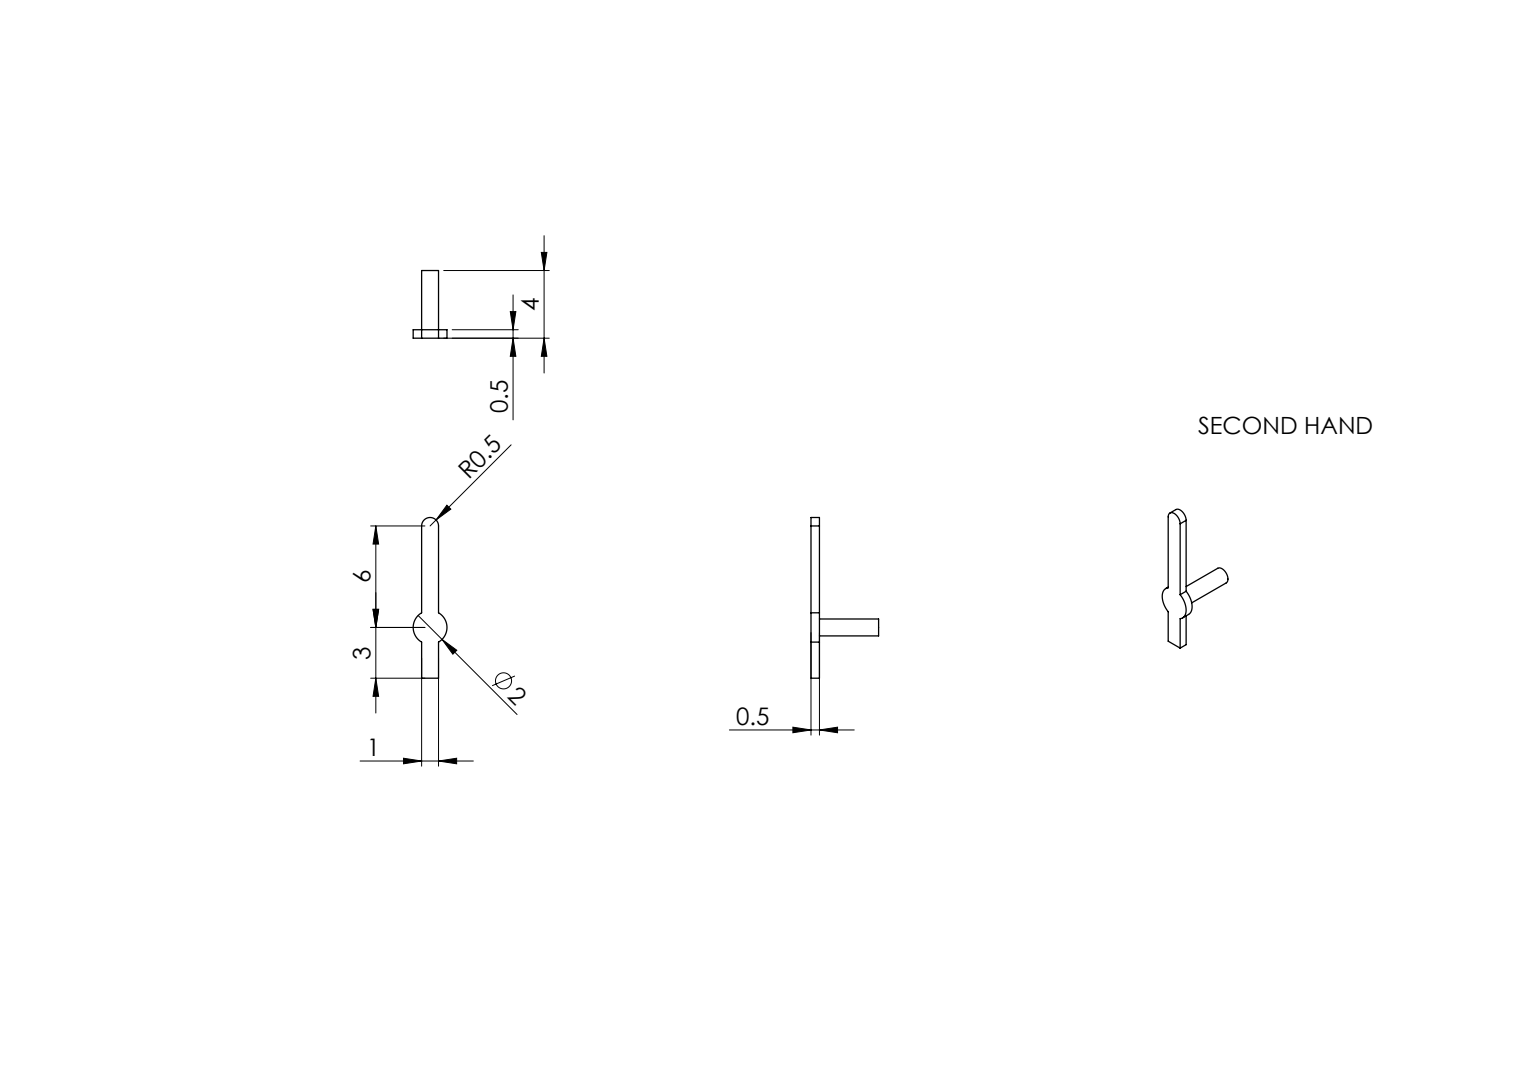
ISO-10303-21;
HEADER;
FILE_DESCRIPTION (('STEP AP214'),
    '1' );
FILE_NAME ('second hand.step',
    '2026-10-26T11:20:31',
    ( '' ),
    ( '' ),
    'SwSTEP 2.0',
    'SolidWorks 2026',
    '' );
FILE_SCHEMA (( 'AUTOMOTIVE_DESIGN' ));
ENDSEC;

DATA;
#9=FACE_OUTER_BOUND ( 'NONE', #3478, .T. ) ;
#19=CARTESIAN_POINT ( 'NONE',  ( -0.5000000000000000000, -2.999999999999999556, 19.50000000000000000 ) ) ;
#36=AXIS2_PLACEMENT_3D ( 'NONE', #4466, #800, #1180 ) ;
#37=CARTESIAN_POINT ( 'NONE',  ( 0.5000000000000001110, 6.123233995736767268E-17, 20.00000000000000000 ) ) ;
#46=ORIENTED_EDGE ( 'NONE', *, *, #3772, .T. ) ;
#54=EDGE_CURVE ( 'NONE', #3353, #742, #2591, .T. ) ;
#56=DIRECTION ( 'NONE',  ( 1.000000000000000000, 0.000000000000000000, -0.000000000000000000 ) ) ;
#58=CARTESIAN_POINT ( 'NONE',  ( -0.5000000000000000000, 0.000000000000000000, 20.00000000000000000 ) ) ;
#60=ORIENTED_EDGE ( 'NONE', *, *, #514, .T. ) ;
#93=PLANE ( 'NONE',  #36 ) ;
#95=ORIENTED_EDGE ( 'NONE', *, *, #3675, .F. ) ;
#128=CARTESIAN_POINT ( 'NONE',  ( -0.5000000000000000000, -2.999999999999999556, 20.00000000000000000 ) ) ;
#137=DIRECTION ( 'NONE',  ( 0.000000000000000000, 0.000000000000000000, 1.000000000000000000 ) ) ;
#163=DIRECTION ( 'NONE',  ( -0.000000000000000000, -1.000000000000000000, 0.000000000000000000 ) ) ;
#177=VERTEX_POINT ( 'NONE', #3882 ) ;
#192=ORIENTED_EDGE ( 'NONE', *, *, #766, .F. ) ;
#197=VECTOR ( 'NONE', #3332, 1000.000000000000000 ) ;
#198=EDGE_CURVE ( 'NONE', #954, #442, #3903, .T. ) ;
#199=EDGE_CURVE ( 'NONE', #177, #2707, #3976, .T. ) ;
#209=CARTESIAN_POINT ( 'NONE',  ( 1.000000000000000000, 0.000000000000000000, 20.00000000000000000 ) ) ;
#216=ORIENTED_EDGE ( 'NONE', *, *, #4488, .T. ) ;
#225=AXIS2_PLACEMENT_3D ( 'NONE', #2885, #1132, #2148 ) ;
#232=CARTESIAN_POINT ( 'NONE',  ( -0.5000000000000000000, 0.000000000000000000, 19.50000000000000000 ) ) ;
#249=ORIENTED_EDGE ( 'NONE', *, *, #4128, .F. ) ;
#252=PLANE ( 'NONE',  #505 ) ;
#279=LINE ( 'NONE', #643, #686 ) ;
#281=EDGE_CURVE ( 'NONE', #1290, #3612, #2017, .T. ) ;
#296=AXIS2_PLACEMENT_3D ( 'NONE', #2408, #3159, #4617 ) ;
#302=CARTESIAN_POINT ( 'NONE',  ( 0.000000000000000000, 0.000000000000000000, 16.00000000000000000 ) ) ;
#312=ADVANCED_FACE ( 'NONE', ( #2776 ), #4236, .F. ) ;
#322=AXIS2_PLACEMENT_3D ( 'NONE', #4183, #3766, #484 ) ;
#326=EDGE_LOOP ( 'NONE', ( #3897, #833, #3483, #60 ) ) ;
#329=SURFACE_SIDE_STYLE ('',( #2159 ) ) ;
#330=DIRECTION ( 'NONE',  ( -1.000000000000000000, 0.000000000000000000, -0.000000000000000000 ) ) ;
#337=AXIS2_PLACEMENT_3D ( 'NONE', #302, #2550, #4345 ) ;
#348=CARTESIAN_POINT ( 'NONE',  ( -0.5000000000000000000, -0.8660254037844387076, 19.50000000000000000 ) ) ;
#355=ORIENTED_EDGE ( 'NONE', *, *, #1156, .F. ) ;
#375=DIRECTION ( 'NONE',  ( 0.000000000000000000, 0.000000000000000000, 1.000000000000000000 ) ) ;
#382=FACE_OUTER_BOUND ( 'NONE', #909, .T. ) ;
#384=CARTESIAN_POINT ( 'NONE',  ( 0.5000000000000000000, 0.000000000000000000, 19.50000000000000000 ) ) ;
#404=SHAPE_REPRESENTATION ( 'second hand', ( #2928 ), #3465 ) ;
#423=CYLINDRICAL_SURFACE ( 'NONE', #4197, 1.000000000000000000 ) ;
#424=EDGE_LOOP ( 'NONE', ( #1754, #498 ) ) ;
#434=ORIENTED_EDGE ( 'NONE', *, *, #4128, .T. ) ;
#442=VERTEX_POINT ( 'NONE', #348 ) ;
#454=CARTESIAN_POINT ( 'NONE',  ( -0.5000000000000001110, 0.000000000000000000, 16.00000000000000000 ) ) ;
#461=CARTESIAN_POINT ( 'NONE',  ( -0.5000000000000000000, 6.000000000000000000, 19.50000000000000000 ) ) ;
#464=CARTESIAN_POINT ( 'NONE',  ( 0.5000000000000000000, -2.999999999999999556, 19.50000000000000000 ) ) ;
#466=DIRECTION ( 'NONE',  ( 1.000000000000000000, 0.000000000000000000, -0.000000000000000000 ) ) ;
#472=VECTOR ( 'NONE', #1598, 1000.000000000000000 ) ;
#474=FACE_OUTER_BOUND ( 'NONE', #326, .T. ) ;
#484=DIRECTION ( 'NONE',  ( 1.000000000000000000, 0.000000000000000000, 0.000000000000000000 ) ) ;
#498=ORIENTED_EDGE ( 'NONE', *, *, #3330, .T. ) ;
#499=VERTEX_POINT ( 'NONE', #19 ) ;
#505=AXIS2_PLACEMENT_3D ( 'NONE', #4213, #3849, #899 ) ;
#514=EDGE_CURVE ( 'NONE', #3612, #442, #4534, .T. ) ;
#527=VECTOR ( 'NONE', #1706, 1000.000000000000000 ) ;
#553=CIRCLE ( 'NONE', #2066, 1.000000000000000000 ) ;
#555=( NAMED_UNIT ( * ) SI_UNIT ( $, .STERADIAN. ) SOLID_ANGLE_UNIT ( ) );
#557=VECTOR ( 'NONE', #4315, 1000.000000000000000 ) ;
#575=LINE ( 'NONE', #4261, #2798 ) ;
#603=ADVANCED_FACE ( 'NONE', ( #1206 ), #2987, .F. ) ;
#643=CARTESIAN_POINT ( 'NONE',  ( 0.5000000000000000000, 0.000000000000000000, 20.00000000000000000 ) ) ;
#654=DIRECTION ( 'NONE',  ( 0.000000000000000000, 0.000000000000000000, 1.000000000000000000 ) ) ;
#673=DIRECTION ( 'NONE',  ( -0.000000000000000000, 0.000000000000000000, 1.000000000000000000 ) ) ;
#686=VECTOR ( 'NONE', #1993, 1000.000000000000000 ) ;
#689=FACE_OUTER_BOUND ( 'NONE', #2400, .T. ) ;
#691=DIRECTION ( 'NONE',  ( 1.000000000000000000, 0.000000000000000000, 0.000000000000000000 ) ) ;
#725=CARTESIAN_POINT ( 'NONE',  ( -0.5000000000000000000, 0.000000000000000000, 19.50000000000000000 ) ) ;
#726=DIRECTION ( 'NONE',  ( 1.000000000000000000, 0.000000000000000000, 0.000000000000000000 ) ) ;
#727=EDGE_CURVE ( 'NONE', #442, #499, #2378, .T. ) ;
#736=ORIENTED_EDGE ( 'NONE', *, *, #2437, .F. ) ;
#737=EDGE_LOOP ( 'NONE', ( #3427, #3754, #3126, #2585 ) ) ;
#742=VERTEX_POINT ( 'NONE', #209 ) ;
#751=EDGE_CURVE ( 'NONE', #954, #2636, #2353, .T. ) ;
#766=EDGE_CURVE ( 'NONE', #1507, #1468, #1480, .T. ) ;
#791=CARTESIAN_POINT ( 'NONE',  ( 0.000000000000000000, 6.000000000000000000, 19.50000000000000000 ) ) ;
#792=CARTESIAN_POINT ( 'NONE',  ( 0.5000000000000001110, 6.123233995736767268E-17, 16.00000000000000000 ) ) ;
#795=PLANE ( 'NONE',  #1205 ) ;
#798=MECHANICAL_DESIGN_GEOMETRIC_PRESENTATION_REPRESENTATION('',(#3759),#4070);
#800=DIRECTION ( 'NONE',  ( 0.000000000000000000, 0.000000000000000000, 1.000000000000000000 ) ) ;
#803=VERTEX_POINT ( 'NONE', #3872 ) ;
#807=ADVANCED_FACE ( 'NONE', ( #2697 ), #252, .T. ) ;
#818=DIRECTION ( 'NONE',  ( -0.000000000000000000, -0.000000000000000000, -1.000000000000000000 ) ) ;
#831=CARTESIAN_POINT ( 'NONE',  ( 0.000000000000000000, 0.000000000000000000, 19.50000000000000000 ) ) ;
#832=CARTESIAN_POINT ( 'NONE',  ( 0.5000000000000000000, 0.000000000000000000, 19.50000000000000000 ) ) ;
#833=ORIENTED_EDGE ( 'NONE', *, *, #2217, .F. ) ;
#841=LINE ( 'NONE', #58, #197 ) ;
#861=AXIS2_PLACEMENT_3D ( 'NONE', #1053, #2489, #4334 ) ;
#862=DIRECTION ( 'NONE',  ( 0.000000000000000000, 0.000000000000000000, 1.000000000000000000 ) ) ;
#892=LINE ( 'NONE', #4485, #4501 ) ;
#895=VERTEX_POINT ( 'NONE', #792 ) ;
#899=DIRECTION ( 'NONE',  ( -0.000000000000000000, 0.000000000000000000, 1.000000000000000000 ) ) ;
#909=EDGE_LOOP ( 'NONE', ( #4375, #2617, #4238, #1805 ) ) ;
#915=DIRECTION ( 'NONE',  ( -0.000000000000000000, -0.000000000000000000, -1.000000000000000000 ) ) ;
#928=PRODUCT_DEFINITION_SHAPE ( 'NONE', 'NONE',  #2893 ) ;
#937=AXIS2_PLACEMENT_3D ( 'NONE', #2131, #1063, #2405 ) ;
#954=VERTEX_POINT ( 'NONE', #1825 ) ;
#959=CARTESIAN_POINT ( 'NONE',  ( 0.5000000000000000000, 0.8660254037844387076, 19.50000000000000000 ) ) ;
#980=ORIENTED_EDGE ( 'NONE', *, *, #281, .F. ) ;
#992=ORIENTED_EDGE ( 'NONE', *, *, #4436, .T. ) ;
#999=ORIENTED_EDGE ( 'NONE', *, *, #1043, .F. ) ;
#1025=( LENGTH_UNIT ( ) NAMED_UNIT ( * ) SI_UNIT ( .MILLI., .METRE. ) );
#1038=AXIS2_PLACEMENT_3D ( 'NONE', #4283, #2088, #691 ) ;
#1043=EDGE_CURVE ( 'NONE', #177, #742, #2922, .T. ) ;
#1047=ORIENTED_EDGE ( 'NONE', *, *, #2083, .T. ) ;
#1050=( NAMED_UNIT ( * ) PLANE_ANGLE_UNIT ( ) SI_UNIT ( $, .RADIAN. ) );
#1053=CARTESIAN_POINT ( 'NONE',  ( 0.000000000000000000, 0.000000000000000000, 19.50000000000000000 ) ) ;
#1054=AXIS2_PLACEMENT_3D ( 'NONE', #725, #2166, #1235 ) ;
#1062=CIRCLE ( 'NONE', #4402, 0.5000000000000001110 ) ;
#1063=DIRECTION ( 'NONE',  ( 0.000000000000000000, 0.000000000000000000, 1.000000000000000000 ) ) ;
#1080=CARTESIAN_POINT ( 'NONE',  ( 0.000000000000000000, 6.000000000000000000, 20.00000000000000000 ) ) ;
#1101=DIRECTION ( 'NONE',  ( 0.000000000000000000, 0.000000000000000000, 1.000000000000000000 ) ) ;
#1123=ORIENTED_EDGE ( 'NONE', *, *, #514, .F. ) ;
#1127=DIRECTION ( 'NONE',  ( 0.000000000000000000, 0.000000000000000000, 1.000000000000000000 ) ) ;
#1132=DIRECTION ( 'NONE',  ( -0.000000000000000000, -0.000000000000000000, -1.000000000000000000 ) ) ;
#1139=VECTOR ( 'NONE', #3148, 1000.000000000000000 ) ;
#1140=CARTESIAN_POINT ( 'NONE',  ( 0.000000000000000000, 0.000000000000000000, 16.00000000000000000 ) ) ;
#1141=ORIENTED_EDGE ( 'NONE', *, *, #2112, .F. ) ;
#1156=EDGE_CURVE ( 'NONE', #2707, #1507, #2249, .T. ) ;
#1180=DIRECTION ( 'NONE',  ( 1.000000000000000000, 0.000000000000000000, -0.000000000000000000 ) ) ;
#1181=ADVANCED_FACE ( 'NONE', ( #474 ), #423, .T. ) ;
#1187=DIRECTION ( 'NONE',  ( 0.000000000000000000, 0.000000000000000000, 1.000000000000000000 ) ) ;
#1200=DIRECTION ( 'NONE',  ( 0.000000000000000000, 0.000000000000000000, 1.000000000000000000 ) ) ;
#1201=CARTESIAN_POINT ( 'NONE',  ( -0.5000000000000001110, 0.000000000000000000, 20.00000000000000000 ) ) ;
#1205=AXIS2_PLACEMENT_3D ( 'NONE', #384, #4363, #1860 ) ;
#1206=FACE_OUTER_BOUND ( 'NONE', #2386, .T. ) ;
#1233=VECTOR ( 'NONE', #1200, 1000.000000000000000 ) ;
#1235=DIRECTION ( 'NONE',  ( 0.000000000000000000, 0.000000000000000000, 1.000000000000000000 ) ) ;
#1275=ADVANCED_FACE ( 'NONE', ( #3542 ), #2875, .F. ) ;
#1276=FACE_OUTER_BOUND ( 'NONE', #1397, .T. ) ;
#1290=VERTEX_POINT ( 'NONE', #3070 ) ;
#1300=DIRECTION ( 'NONE',  ( -1.000000000000000000, 0.000000000000000000, 0.000000000000000000 ) ) ;
#1301=LINE ( 'NONE', #4557, #2188 ) ;
#1303=ORIENTED_EDGE ( 'NONE', *, *, #1916, .T. ) ;
#1307=CARTESIAN_POINT ( 'NONE',  ( 0.000000000000000000, 6.000000000000000000, 19.50000000000000000 ) ) ;
#1318=VECTOR ( 'NONE', #137, 1000.000000000000000 ) ;
#1355=CARTESIAN_POINT ( 'NONE',  ( 0.000000000000000000, 0.000000000000000000, 19.50000000000000000 ) ) ;
#1390=AXIS2_PLACEMENT_3D ( 'NONE', #3409, #915, #1300 ) ;
#1397=EDGE_LOOP ( 'NONE', ( #999, #2989, #3673, #2512 ) ) ;
#1441=EDGE_LOOP ( 'NONE', ( #46, #1980, #4001, #3042 ) ) ;
#1444=CARTESIAN_POINT ( 'NONE',  ( -0.5000000000000000000, 6.000000000000000000, 19.50000000000000000 ) ) ;
#1452=DIRECTION ( 'NONE',  ( 1.000000000000000000, 0.000000000000000000, 0.000000000000000000 ) ) ;
#1454=FACE_OUTER_BOUND ( 'NONE', #2925, .T. ) ;
#1468=VERTEX_POINT ( 'NONE', #1444 ) ;
#1476=CYLINDRICAL_SURFACE ( 'NONE', #225, 0.5000000000000001110 ) ;
#1480=CIRCLE ( 'NONE', #4233, 0.5000000000000000000 ) ;
#1498=EDGE_LOOP ( 'NONE', ( #4018, #1047, #3591, #736 ) ) ;
#1499=LINE ( 'NONE', #37, #3410 ) ;
#1507=VERTEX_POINT ( 'NONE', #2528 ) ;
#1524=EDGE_CURVE ( 'NONE', #4308, #3204, #1923, .T. ) ;
#1552=LINE ( 'NONE', #461, #472 ) ;
#1559=COLOUR_RGB ( '',0.8941176470588234615, 0.8941176470588234615, 0.8941176470588234615 ) ;
#1563=DIRECTION ( 'NONE',  ( 1.000000000000000000, 0.000000000000000000, 0.000000000000000000 ) ) ;
#1598=DIRECTION ( 'NONE',  ( 0.000000000000000000, 0.000000000000000000, 1.000000000000000000 ) ) ;
#1614=VERTEX_POINT ( 'NONE', #3113 ) ;
#1629=CARTESIAN_POINT ( 'NONE',  ( -0.5000000000000000000, 0.000000000000000000, 20.00000000000000000 ) ) ;
#1642=( LENGTH_UNIT ( ) NAMED_UNIT ( * ) SI_UNIT ( .MILLI., .METRE. ) );
#1646=DIRECTION ( 'NONE',  ( 1.000000000000000000, 0.000000000000000000, 0.000000000000000000 ) ) ;
#1660=EDGE_LOOP ( 'NONE', ( #3022, #4009, #2737, #3858 ) ) ;
#1679=CYLINDRICAL_SURFACE ( 'NONE', #937, 1.000000000000000000 ) ;
#1702=ADVANCED_FACE ( 'NONE', ( #689 ), #1679, .T. ) ;
#1706=DIRECTION ( 'NONE',  ( -0.000000000000000000, -0.000000000000000000, -1.000000000000000000 ) ) ;
#1707=AXIS2_PLACEMENT_3D ( 'NONE', #791, #1127, #1452 ) ;
#1712=DIRECTION ( 'NONE',  ( 0.000000000000000000, 0.000000000000000000, 1.000000000000000000 ) ) ;
#1725=EDGE_CURVE ( 'NONE', #803, #177, #553, .T. ) ;
#1754=ORIENTED_EDGE ( 'NONE', *, *, #3245, .T. ) ;
#1778=SURFACE_STYLE_USAGE ( .BOTH. , #329 ) ;
#1780=CARTESIAN_POINT ( 'NONE',  ( 0.000000000000000000, 0.000000000000000000, 0.000000000000000000 ) ) ;
#1798=ORIENTED_EDGE ( 'NONE', *, *, #2943, .T. ) ;
#1805=ORIENTED_EDGE ( 'NONE', *, *, #2112, .T. ) ;
#1825=CARTESIAN_POINT ( 'NONE',  ( -0.5000000000000000000, -0.8660254037844387076, 20.00000000000000000 ) ) ;
#1835=ORIENTED_EDGE ( 'NONE', *, *, #3330, .F. ) ;
#1860=DIRECTION ( 'NONE',  ( 0.000000000000000000, 0.000000000000000000, -1.000000000000000000 ) ) ;
#1896=VERTEX_POINT ( 'NONE', #3604 ) ;
#1898=CARTESIAN_POINT ( 'NONE',  ( 0.5000000000000000000, -2.999999999999999556, 19.50000000000000000 ) ) ;
#1905=EDGE_LOOP ( 'NONE', ( #980, #2055, #1141, #3288 ) ) ;
#1909=CARTESIAN_POINT ( 'NONE',  ( -0.5000000000000001110, 0.000000000000000000, 19.50000000000000000 ) ) ;
#1916=EDGE_CURVE ( 'NONE', #4308, #499, #1919, .T. ) ;
#1919=LINE ( 'NONE', #464, #3360 ) ;
#1923=LINE ( 'NONE', #1898, #2655 ) ;
#1927=ORIENTED_EDGE ( 'NONE', *, *, #751, .T. ) ;
#1937=FACE_OUTER_BOUND ( 'NONE', #2766, .T. ) ;
#1964=DIRECTION ( 'NONE',  ( 0.000000000000000000, 0.000000000000000000, 1.000000000000000000 ) ) ;
#1980=ORIENTED_EDGE ( 'NONE', *, *, #2095, .F. ) ;
#1993=DIRECTION ( 'NONE',  ( 0.000000000000000000, 1.000000000000000000, 0.000000000000000000 ) ) ;
#2017=LINE ( 'NONE', #2361, #527 ) ;
#2041=AXIS2_PLACEMENT_3D ( 'NONE', #4358, #1101, #56 ) ;
#2055=ORIENTED_EDGE ( 'NONE', *, *, #4488, .F. ) ;
#2057=EDGE_CURVE ( 'NONE', #1507, #1896, #2282, .T. ) ;
#2066=AXIS2_PLACEMENT_3D ( 'NONE', #1355, #4590, #3894 ) ;
#2075=FACE_OUTER_BOUND ( 'NONE', #1905, .T. ) ;
#2077=ORIENTED_EDGE ( 'NONE', *, *, #2217, .T. ) ;
#2083=EDGE_CURVE ( 'NONE', #3353, #3204, #892, .T. ) ;
#2088=DIRECTION ( 'NONE',  ( 0.000000000000000000, 0.000000000000000000, 1.000000000000000000 ) ) ;
#2095=EDGE_CURVE ( 'NONE', #499, #2636, #4508, .T. ) ;
#2112=EDGE_CURVE ( 'NONE', #1468, #2610, #1552, .T. ) ;
#2124=LINE ( 'NONE', #3570, #1139 ) ;
#2131=CARTESIAN_POINT ( 'NONE',  ( 0.000000000000000000, 0.000000000000000000, 19.50000000000000000 ) ) ;
#2137=FILL_AREA_STYLE ('',( #4624 ) ) ;
#2148=DIRECTION ( 'NONE',  ( -1.000000000000000000, 0.000000000000000000, 0.000000000000000000 ) ) ;
#2157=VECTOR ( 'NONE', #4063, 1000.000000000000000 ) ;
#2159=SURFACE_STYLE_FILL_AREA ( #2137 ) ;
#2166=DIRECTION ( 'NONE',  ( -1.000000000000000000, 0.000000000000000000, 0.000000000000000000 ) ) ;
#2168=ADVANCED_FACE ( 'NONE', ( #1276 ), #2716, .T. ) ;
#2171=AXIS2_PLACEMENT_3D ( 'NONE', #1140, #4441, #466 ) ;
#2188=VECTOR ( 'NONE', #3101, 1000.000000000000000 ) ;
#2191=EDGE_CURVE ( 'NONE', #742, #1614, #4665, .T. ) ;
#2192=ADVANCED_FACE ( 'NONE', ( #1937 ), #3385, .T. ) ;
#2197=VECTOR ( 'NONE', #4423, 1000.000000000000000 ) ;
#2211=CIRCLE ( 'NONE', #2829, 1.000000000000000000 ) ;
#2217=EDGE_CURVE ( 'NONE', #1290, #954, #2211, .T. ) ;
#2228=LINE ( 'NONE', #3261, #3792 ) ;
#2249=LINE ( 'NONE', #832, #2197 ) ;
#2254=UNCERTAINTY_MEASURE_WITH_UNIT (LENGTH_MEASURE( 1.000000000000000082E-05 ), #1642, 'distance_accuracy_value', 'NONE');
#2282=LINE ( 'NONE', #2689, #1318 ) ;
#2310=DIRECTION ( 'NONE',  ( -0.000000000000000000, -1.000000000000000000, 0.000000000000000000 ) ) ;
#2353=LINE ( 'NONE', #1629, #2390 ) ;
#2361=CARTESIAN_POINT ( 'NONE',  ( -0.5000000000000000000, 0.8660254037844387076, 19.50000000000000000 ) ) ;
#2371=DIRECTION ( 'NONE',  ( 0.000000000000000000, 0.000000000000000000, 1.000000000000000000 ) ) ;
#2378=LINE ( 'NONE', #232, #3536 ) ;
#2386=EDGE_LOOP ( 'NONE', ( #4145, #95 ) ) ;
#2390=VECTOR ( 'NONE', #2310, 1000.000000000000000 ) ;
#2399=CARTESIAN_POINT ( 'NONE',  ( 0.5000000000000000000, -2.999999999999999556, 19.50000000000000000 ) ) ;
#2400=EDGE_LOOP ( 'NONE', ( #3401, #2896, #2815, #3828 ) ) ;
#2405=DIRECTION ( 'NONE',  ( 1.000000000000000000, 0.000000000000000000, 0.000000000000000000 ) ) ;
#2408=CARTESIAN_POINT ( 'NONE',  ( 0.5000000000000000000, -2.999999999999999556, 19.50000000000000000 ) ) ;
#2414=SHAPE_REPRESENTATION_RELATIONSHIP ( 'NONE' , 'NONE' ,  #404, #4678 ) ;
#2437=EDGE_CURVE ( 'NONE', #803, #4308, #2228, .T. ) ;
#2458=ORIENTED_EDGE ( 'NONE', *, *, #199, .F. ) ;
#2480=ADVANCED_FACE ( 'NONE', ( #9, #2906 ), #4316, .F. ) ;
#2489=DIRECTION ( 'NONE',  ( 0.000000000000000000, 0.000000000000000000, 1.000000000000000000 ) ) ;
#2506=ORIENTED_EDGE ( 'NONE', *, *, #727, .F. ) ;
#2512=ORIENTED_EDGE ( 'NONE', *, *, #2191, .F. ) ;
#2525=ORIENTED_EDGE ( 'NONE', *, *, #2437, .T. ) ;
#2528=CARTESIAN_POINT ( 'NONE',  ( 0.5000000000000000000, 6.000000000000000000, 19.50000000000000000 ) ) ;
#2550=DIRECTION ( 'NONE',  ( 0.000000000000000000, 0.000000000000000000, 1.000000000000000000 ) ) ;
#2568=CIRCLE ( 'NONE', #4175, 0.5000000000000001110 ) ;
#2571=LINE ( 'NONE', #1201, #4143 ) ;
#2577=VERTEX_POINT ( 'NONE', #454 ) ;
#2585=ORIENTED_EDGE ( 'NONE', *, *, #2095, .T. ) ;
#2591=CIRCLE ( 'NONE', #3801, 1.000000000000000000 ) ;
#2607=DIRECTION ( 'NONE',  ( 1.000000000000000000, 0.000000000000000000, 0.000000000000000000 ) ) ;
#2610=VERTEX_POINT ( 'NONE', #4147 ) ;
#2617=ORIENTED_EDGE ( 'NONE', *, *, #2057, .F. ) ;
#2619=CARTESIAN_POINT ( 'NONE',  ( -0.5000000000000000000, -2.999999999999999556, 19.50000000000000000 ) ) ;
#2621=STYLED_ITEM ( 'NONE', ( #3901 ), #4678 ) ;
#2636=VERTEX_POINT ( 'NONE', #128 ) ;
#2655=VECTOR ( 'NONE', #3346, 1000.000000000000000 ) ;
#2663=( NAMED_UNIT ( * ) PLANE_ANGLE_UNIT ( ) SI_UNIT ( $, .RADIAN. ) );
#2670=AXIS2_PLACEMENT_3D ( 'NONE', #3817, #1964, #1646 ) ;
#2677=ORIENTED_EDGE ( 'NONE', *, *, #1725, .F. ) ;
#2689=CARTESIAN_POINT ( 'NONE',  ( 0.5000000000000000000, 6.000000000000000000, 19.50000000000000000 ) ) ;
#2697=FACE_OUTER_BOUND ( 'NONE', #737, .T. ) ;
#2707=VERTEX_POINT ( 'NONE', #959 ) ;
#2715=EDGE_CURVE ( 'NONE', #1468, #3612, #575, .T. ) ;
#2716=CYLINDRICAL_SURFACE ( 'NONE', #322, 1.000000000000000000 ) ;
#2737=ORIENTED_EDGE ( 'NONE', *, *, #2057, .T. ) ;
#2743=EDGE_LOOP ( 'NONE', ( #2077, #1927, #2923, #3559, #4122, #3446, #3707, #992, #216 ) ) ;
#2766=EDGE_LOOP ( 'NONE', ( #2970, #3747, #434, #4042 ) ) ;
#2776=FACE_OUTER_BOUND ( 'NONE', #1441, .T. ) ;
#2786=( NAMED_UNIT ( * ) PLANE_ANGLE_UNIT ( ) SI_UNIT ( $, .RADIAN. ) );
#2795=APPLICATION_CONTEXT ( 'automotive_design' ) ;
#2798=VECTOR ( 'NONE', #2805, 1000.000000000000000 ) ;
#2805=DIRECTION ( 'NONE',  ( -0.000000000000000000, -1.000000000000000000, -0.000000000000000000 ) ) ;
#2815=ORIENTED_EDGE ( 'NONE', *, *, #54, .F. ) ;
#2822=CARTESIAN_POINT ( 'NONE',  ( -0.5000000000000000000, 0.8660254037844387076, 19.50000000000000000 ) ) ;
#2829=AXIS2_PLACEMENT_3D ( 'NONE', #3883, #2371, #4205 ) ;
#2855=CARTESIAN_POINT ( 'NONE',  ( -0.5000000000000000000, -0.8660254037844387076, 19.50000000000000000 ) ) ;
#2875=PLANE ( 'NONE',  #3764 ) ;
#2885=CARTESIAN_POINT ( 'NONE',  ( 0.000000000000000000, 0.000000000000000000, 20.00000000000000000 ) ) ;
#2893=PRODUCT_DEFINITION ( 'UNKNOWN', '', #3312, #4290 ) ;
#2896=ORIENTED_EDGE ( 'NONE', *, *, #1043, .T. ) ;
#2906=FACE_BOUND ( 'NONE', #424, .T. ) ;
#2914=CIRCLE ( 'NONE', #337, 0.5000000000000001110 ) ;
#2922=LINE ( 'NONE', #4374, #3776 ) ;
#2923=ORIENTED_EDGE ( 'NONE', *, *, #3772, .F. ) ;
#2925=EDGE_LOOP ( 'NONE', ( #1835, #1798, #3614, #249 ) ) ;
#2928=AXIS2_PLACEMENT_3D ( 'NONE', #1780, #1712, #3957 ) ;
#2933=( GEOMETRIC_REPRESENTATION_CONTEXT ( 3 ) GLOBAL_UNCERTAINTY_ASSIGNED_CONTEXT ( ( #3048 ) ) GLOBAL_UNIT_ASSIGNED_CONTEXT ( ( #1025, #2786, #3256 ) ) REPRESENTATION_CONTEXT ( 'NONE', 'WORKASPACE' ) );
#2935=DIRECTION ( 'NONE',  ( -0.000000000000000000, -0.000000000000000000, -1.000000000000000000 ) ) ;
#2939=ADVANCED_FACE ( 'NONE', ( #4056 ), #795, .T. ) ;
#2943=EDGE_CURVE ( 'NONE', #4217, #895, #1499, .T. ) ;
#2958=ADVANCED_FACE ( 'NONE', ( #1454 ), #1476, .T. ) ;
#2970=ORIENTED_EDGE ( 'NONE', *, *, #2943, .F. ) ;
#2987=PLANE ( 'NONE',  #2171 ) ;
#2989=ORIENTED_EDGE ( 'NONE', *, *, #199, .T. ) ;
#3022=ORIENTED_EDGE ( 'NONE', *, *, #3074, .F. ) ;
#3034=FACE_OUTER_BOUND ( 'NONE', #2743, .T. ) ;
#3042=ORIENTED_EDGE ( 'NONE', *, *, #1524, .T. ) ;
#3048=UNCERTAINTY_MEASURE_WITH_UNIT (LENGTH_MEASURE( 1.000000000000000082E-05 ), #1025, 'distance_accuracy_value', 'NONE');
#3070=CARTESIAN_POINT ( 'NONE',  ( -0.5000000000000000000, 0.8660254037844387076, 20.00000000000000000 ) ) ;
#3074=EDGE_CURVE ( 'NONE', #2707, #1614, #1301, .T. ) ;
#3101=DIRECTION ( 'NONE',  ( 0.000000000000000000, 0.000000000000000000, 1.000000000000000000 ) ) ;
#3113=CARTESIAN_POINT ( 'NONE',  ( 0.5000000000000000000, 0.8660254037844387076, 20.00000000000000000 ) ) ;
#3126=ORIENTED_EDGE ( 'NONE', *, *, #727, .T. ) ;
#3148=DIRECTION ( 'NONE',  ( -0.000000000000000000, -0.000000000000000000, -1.000000000000000000 ) ) ;
#3151=CIRCLE ( 'NONE', #4366, 0.5000000000000000000 ) ;
#3159=DIRECTION ( 'NONE',  ( 0.000000000000000000, 1.000000000000000000, -0.000000000000000000 ) ) ;
#3160=EDGE_CURVE ( 'NONE', #3353, #803, #2124, .T. ) ;
#3204=VERTEX_POINT ( 'NONE', #4604 ) ;
#3208=( NAMED_UNIT ( * ) SI_UNIT ( $, .STERADIAN. ) SOLID_ANGLE_UNIT ( ) );
#3245=EDGE_CURVE ( 'NONE', #4522, #4217, #2568, .T. ) ;
#3256=( NAMED_UNIT ( * ) SI_UNIT ( $, .STERADIAN. ) SOLID_ANGLE_UNIT ( ) );
#3261=CARTESIAN_POINT ( 'NONE',  ( 0.5000000000000000000, 0.000000000000000000, 19.50000000000000000 ) ) ;
#3288=ORIENTED_EDGE ( 'NONE', *, *, #2715, .T. ) ;
#3299=ADVANCED_FACE ( 'NONE', ( #2075 ), #3546, .T. ) ;
#3312=PRODUCT_DEFINITION_FORMATION_WITH_SPECIFIED_SOURCE ( 'ANY', '', #3390, .NOT_KNOWN. ) ;
#3320=ORIENTED_EDGE ( 'NONE', *, *, #2715, .F. ) ;
#3330=EDGE_CURVE ( 'NONE', #4217, #4522, #1062, .T. ) ;
#3332=DIRECTION ( 'NONE',  ( -0.000000000000000000, -1.000000000000000000, -0.000000000000000000 ) ) ;
#3346=DIRECTION ( 'NONE',  ( 0.000000000000000000, 0.000000000000000000, 1.000000000000000000 ) ) ;
#3353=VERTEX_POINT ( 'NONE', #4006 ) ;
#3360=VECTOR ( 'NONE', #3365, 1000.000000000000000 ) ;
#3365=DIRECTION ( 'NONE',  ( -1.000000000000000000, 0.000000000000000000, 0.000000000000000000 ) ) ;
#3385=CYLINDRICAL_SURFACE ( 'NONE', #1390, 0.5000000000000001110 ) ;
#3390=PRODUCT ( 'second hand', 'second hand', '', ( #3646 ) ) ;
#3392=EDGE_CURVE ( 'NONE', #2577, #895, #4561, .T. ) ;
#3399=DIRECTION ( 'NONE',  ( 1.000000000000000000, 0.000000000000000000, 0.000000000000000000 ) ) ;
#3401=ORIENTED_EDGE ( 'NONE', *, *, #1725, .T. ) ;
#3409=CARTESIAN_POINT ( 'NONE',  ( 0.000000000000000000, 0.000000000000000000, 20.00000000000000000 ) ) ;
#3410=VECTOR ( 'NONE', #2935, 1000.000000000000000 ) ;
#3427=ORIENTED_EDGE ( 'NONE', *, *, #751, .F. ) ;
#3446=ORIENTED_EDGE ( 'NONE', *, *, #2191, .T. ) ;
#3455=DIRECTION ( 'NONE',  ( 1.000000000000000000, 0.000000000000000000, 0.000000000000000000 ) ) ;
#3465=( GEOMETRIC_REPRESENTATION_CONTEXT ( 3 ) GLOBAL_UNCERTAINTY_ASSIGNED_CONTEXT ( ( #4482 ) ) GLOBAL_UNIT_ASSIGNED_CONTEXT ( ( #3954, #1050, #3208 ) ) REPRESENTATION_CONTEXT ( 'NONE', 'WORKASPACE' ) );
#3478=EDGE_LOOP ( 'NONE', ( #2677, #2525, #1303, #2506, #1123, #3320, #192, #355, #2458 ) ) ;
#3480=EDGE_CURVE ( 'NONE', #1614, #1896, #279, .T. ) ;
#3483=ORIENTED_EDGE ( 'NONE', *, *, #281, .T. ) ;
#3536=VECTOR ( 'NONE', #163, 1000.000000000000000 ) ;
#3542=FACE_OUTER_BOUND ( 'NONE', #1498, .T. ) ;
#3546=PLANE ( 'NONE',  #1054 ) ;
#3559=ORIENTED_EDGE ( 'NONE', *, *, #2083, .F. ) ;
#3560=AXIS2_PLACEMENT_3D ( 'NONE', #4448, #1187, #3399 ) ;
#3565=CARTESIAN_POINT ( 'NONE',  ( 0.5000000000000000000, 0.000000000000000000, 19.50000000000000000 ) ) ;
#3570=CARTESIAN_POINT ( 'NONE',  ( 0.5000000000000000000, -0.8660254037844387076, 19.50000000000000000 ) ) ;
#3591=ORIENTED_EDGE ( 'NONE', *, *, #1524, .F. ) ;
#3604=CARTESIAN_POINT ( 'NONE',  ( 0.5000000000000000000, 6.000000000000000000, 20.00000000000000000 ) ) ;
#3612=VERTEX_POINT ( 'NONE', #2822 ) ;
#3614=ORIENTED_EDGE ( 'NONE', *, *, #3675, .T. ) ;
#3646=PRODUCT_CONTEXT ( 'NONE', #2795, 'mechanical' ) ;
#3673=ORIENTED_EDGE ( 'NONE', *, *, #3074, .T. ) ;
#3675=EDGE_CURVE ( 'NONE', #895, #2577, #2914, .T. ) ;
#3683=DIRECTION ( 'NONE',  ( -0.000000000000000000, -1.000000000000000000, 0.000000000000000000 ) ) ;
#3704=CARTESIAN_POINT ( 'NONE',  ( 0.000000000000000000, 0.000000000000000000, 19.50000000000000000 ) ) ;
#3707=ORIENTED_EDGE ( 'NONE', *, *, #3480, .T. ) ;
#3742=DIRECTION ( 'NONE',  ( -0.000000000000000000, -1.000000000000000000, 0.000000000000000000 ) ) ;
#3747=ORIENTED_EDGE ( 'NONE', *, *, #3245, .F. ) ;
#3750=DIRECTION ( 'NONE',  ( 0.000000000000000000, 0.000000000000000000, 1.000000000000000000 ) ) ;
#3754=ORIENTED_EDGE ( 'NONE', *, *, #198, .T. ) ;
#3759=STYLED_ITEM('',(#4757),#4556);
#3764=AXIS2_PLACEMENT_3D ( 'NONE', #3565, #330, #673 ) ;
#3766=DIRECTION ( 'NONE',  ( 0.000000000000000000, 0.000000000000000000, 1.000000000000000000 ) ) ;
#3772=EDGE_CURVE ( 'NONE', #3204, #2636, #4391, .T. ) ;
#3773=ADVANCED_FACE ( 'NONE', ( #3034 ), #93, .T. ) ;
#3776=VECTOR ( 'NONE', #375, 1000.000000000000000 ) ;
#3792=VECTOR ( 'NONE', #3683, 1000.000000000000000 ) ;
#3801=AXIS2_PLACEMENT_3D ( 'NONE', #3816, #862, #3455 ) ;
#3816=CARTESIAN_POINT ( 'NONE',  ( 0.000000000000000000, 0.000000000000000000, 20.00000000000000000 ) ) ;
#3817=CARTESIAN_POINT ( 'NONE',  ( 0.000000000000000000, 0.000000000000000000, 20.00000000000000000 ) ) ;
#3828=ORIENTED_EDGE ( 'NONE', *, *, #3160, .T. ) ;
#3846=MECHANICAL_DESIGN_GEOMETRIC_PRESENTATION_REPRESENTATION('',(#2621),#2933);
#3849=DIRECTION ( 'NONE',  ( -1.000000000000000000, 0.000000000000000000, -0.000000000000000000 ) ) ;
#3858=ORIENTED_EDGE ( 'NONE', *, *, #3480, .F. ) ;
#3872=CARTESIAN_POINT ( 'NONE',  ( 0.5000000000000000000, -0.8660254037844387076, 19.50000000000000000 ) ) ;
#3882=CARTESIAN_POINT ( 'NONE',  ( 1.000000000000000000, 0.000000000000000000, 19.50000000000000000 ) ) ;
#3883=CARTESIAN_POINT ( 'NONE',  ( 0.000000000000000000, 0.000000000000000000, 20.00000000000000000 ) ) ;
#3894=DIRECTION ( 'NONE',  ( 1.000000000000000000, 0.000000000000000000, 0.000000000000000000 ) ) ;
#3897=ORIENTED_EDGE ( 'NONE', *, *, #198, .F. ) ;
#3901=PRESENTATION_STYLE_ASSIGNMENT (( #1778 ) ) ;
#3903=LINE ( 'NONE', #2855, #557 ) ;
#3954=( LENGTH_UNIT ( ) NAMED_UNIT ( * ) SI_UNIT ( .MILLI., .METRE. ) );
#3957=DIRECTION ( 'NONE',  ( 1.000000000000000000, 0.000000000000000000, 0.000000000000000000 ) ) ;
#3976=CIRCLE ( 'NONE', #861, 1.000000000000000000 ) ;
#3984=DIRECTION ( 'NONE',  ( 0.000000000000000000, 0.000000000000000000, 1.000000000000000000 ) ) ;
#4001=ORIENTED_EDGE ( 'NONE', *, *, #1916, .F. ) ;
#4006=CARTESIAN_POINT ( 'NONE',  ( 0.5000000000000000000, -0.8660254037844387076, 20.00000000000000000 ) ) ;
#4009=ORIENTED_EDGE ( 'NONE', *, *, #1156, .T. ) ;
#4018=ORIENTED_EDGE ( 'NONE', *, *, #3160, .F. ) ;
#4042=ORIENTED_EDGE ( 'NONE', *, *, #3392, .T. ) ;
#4044=CLOSED_SHELL ( 'NONE', ( #2958, #1702, #2168, #2192, #3773, #603, #2480, #3299, #4446, #2939, #1181, #807, #1275, #312 ) ) ;
#4056=FACE_OUTER_BOUND ( 'NONE', #1660, .T. ) ;
#4063=DIRECTION ( 'NONE',  ( -1.000000000000000000, 0.000000000000000000, 0.000000000000000000 ) ) ;
#4070=( GEOMETRIC_REPRESENTATION_CONTEXT ( 3 ) GLOBAL_UNCERTAINTY_ASSIGNED_CONTEXT ( ( #2254 ) ) GLOBAL_UNIT_ASSIGNED_CONTEXT ( ( #1642, #2663, #555 ) ) REPRESENTATION_CONTEXT ( 'NONE', 'WORKASPACE' ) );
#4117=DIRECTION ( 'NONE',  ( 0.000000000000000000, 0.000000000000000000, 1.000000000000000000 ) ) ;
#4122=ORIENTED_EDGE ( 'NONE', *, *, #54, .T. ) ;
#4128=EDGE_CURVE ( 'NONE', #4522, #2577, #2571, .T. ) ;
#4143=VECTOR ( 'NONE', #818, 1000.000000000000000 ) ;
#4145=ORIENTED_EDGE ( 'NONE', *, *, #3392, .F. ) ;
#4147=CARTESIAN_POINT ( 'NONE',  ( -0.5000000000000000000, 6.000000000000000000, 20.00000000000000000 ) ) ;
#4166=DIRECTION ( 'NONE',  ( 1.000000000000000000, 0.000000000000000000, 0.000000000000000000 ) ) ;
#4175=AXIS2_PLACEMENT_3D ( 'NONE', #4680, #654, #4295 ) ;
#4183=CARTESIAN_POINT ( 'NONE',  ( 0.000000000000000000, 0.000000000000000000, 19.50000000000000000 ) ) ;
#4197=AXIS2_PLACEMENT_3D ( 'NONE', #3704, #4117, #2607 ) ;
#4205=DIRECTION ( 'NONE',  ( 1.000000000000000000, 0.000000000000000000, 0.000000000000000000 ) ) ;
#4213=CARTESIAN_POINT ( 'NONE',  ( -0.5000000000000000000, 0.000000000000000000, 19.50000000000000000 ) ) ;
#4217=VERTEX_POINT ( 'NONE', #4532 ) ;
#4233=AXIS2_PLACEMENT_3D ( 'NONE', #1307, #4513, #4166 ) ;
#4236=PLANE ( 'NONE',  #296 ) ;
#4238=ORIENTED_EDGE ( 'NONE', *, *, #766, .T. ) ;
#4258=APPLICATION_CONTEXT ( 'automotive_design' ) ;
#4261=CARTESIAN_POINT ( 'NONE',  ( -0.5000000000000000000, 0.000000000000000000, 19.50000000000000000 ) ) ;
#4283=CARTESIAN_POINT ( 'NONE',  ( 0.000000000000000000, 0.000000000000000000, 19.50000000000000000 ) ) ;
#4290=PRODUCT_DEFINITION_CONTEXT ( 'detailed design', #4258, 'design' ) ;
#4295=DIRECTION ( 'NONE',  ( 1.000000000000000000, 0.000000000000000000, 0.000000000000000000 ) ) ;
#4308=VERTEX_POINT ( 'NONE', #2399 ) ;
#4315=DIRECTION ( 'NONE',  ( -0.000000000000000000, -0.000000000000000000, -1.000000000000000000 ) ) ;
#4316=PLANE ( 'NONE',  #2041 ) ;
#4334=DIRECTION ( 'NONE',  ( 1.000000000000000000, 0.000000000000000000, 0.000000000000000000 ) ) ;
#4345=DIRECTION ( 'NONE',  ( 1.000000000000000000, 0.000000000000000000, 0.000000000000000000 ) ) ;
#4358=CARTESIAN_POINT ( 'NONE',  ( 0.000000000000000000, 0.000000000000000000, 19.50000000000000000 ) ) ;
#4363=DIRECTION ( 'NONE',  ( 1.000000000000000000, 0.000000000000000000, 0.000000000000000000 ) ) ;
#4366=AXIS2_PLACEMENT_3D ( 'NONE', #1080, #3984, #726 ) ;
#4374=CARTESIAN_POINT ( 'NONE',  ( 1.000000000000000000, 0.000000000000000000, 19.50000000000000000 ) ) ;
#4375=ORIENTED_EDGE ( 'NONE', *, *, #4436, .F. ) ;
#4385=CYLINDRICAL_SURFACE ( 'NONE', #1707, 0.5000000000000000000 ) ;
#4391=LINE ( 'NONE', #4417, #2157 ) ;
#4402=AXIS2_PLACEMENT_3D ( 'NONE', #831, #3750, #1563 ) ;
#4417=CARTESIAN_POINT ( 'NONE',  ( 0.5000000000000000000, -2.999999999999999556, 20.00000000000000000 ) ) ;
#4423=DIRECTION ( 'NONE',  ( 0.000000000000000000, 1.000000000000000000, 0.000000000000000000 ) ) ;
#4436=EDGE_CURVE ( 'NONE', #1896, #2610, #3151, .T. ) ;
#4441=DIRECTION ( 'NONE',  ( 0.000000000000000000, 0.000000000000000000, 1.000000000000000000 ) ) ;
#4446=ADVANCED_FACE ( 'NONE', ( #382 ), #4385, .T. ) ;
#4448=CARTESIAN_POINT ( 'NONE',  ( 0.000000000000000000, 0.000000000000000000, 16.00000000000000000 ) ) ;
#4466=CARTESIAN_POINT ( 'NONE',  ( 0.000000000000000000, 0.000000000000000000, 20.00000000000000000 ) ) ;
#4482=UNCERTAINTY_MEASURE_WITH_UNIT (LENGTH_MEASURE( 1.000000000000000082E-05 ), #3954, 'distance_accuracy_value', 'NONE');
#4485=CARTESIAN_POINT ( 'NONE',  ( 0.5000000000000000000, 0.000000000000000000, 20.00000000000000000 ) ) ;
#4488=EDGE_CURVE ( 'NONE', #2610, #1290, #841, .T. ) ;
#4501=VECTOR ( 'NONE', #3742, 1000.000000000000000 ) ;
#4508=LINE ( 'NONE', #2619, #1233 ) ;
#4513=DIRECTION ( 'NONE',  ( 0.000000000000000000, 0.000000000000000000, 1.000000000000000000 ) ) ;
#4522=VERTEX_POINT ( 'NONE', #1909 ) ;
#4532=CARTESIAN_POINT ( 'NONE',  ( 0.5000000000000001110, 6.123233995736767268E-17, 19.50000000000000000 ) ) ;
#4534=CIRCLE ( 'NONE', #1038, 1.000000000000000000 ) ;
#4556=MANIFOLD_SOLID_BREP ( 'Extrude-Thin1', #4044 ) ;
#4557=CARTESIAN_POINT ( 'NONE',  ( 0.5000000000000000000, 0.8660254037844387076, 19.50000000000000000 ) ) ;
#4561=CIRCLE ( 'NONE', #3560, 0.5000000000000001110 ) ;
#4590=DIRECTION ( 'NONE',  ( 0.000000000000000000, 0.000000000000000000, 1.000000000000000000 ) ) ;
#4604=CARTESIAN_POINT ( 'NONE',  ( 0.5000000000000000000, -2.999999999999999556, 20.00000000000000000 ) ) ;
#4617=DIRECTION ( 'NONE',  ( 0.000000000000000000, 0.000000000000000000, 1.000000000000000000 ) ) ;
#4624=FILL_AREA_STYLE_COLOUR ( '', #1559 ) ;
#4663=SHAPE_DEFINITION_REPRESENTATION ( #928, #404 ) ;
#4665=CIRCLE ( 'NONE', #2670, 1.000000000000000000 ) ;
#4678=ADVANCED_BREP_SHAPE_REPRESENTATION ( '', ( #4556, #2928 ), #3465 ) ;
#4680=CARTESIAN_POINT ( 'NONE',  ( 0.000000000000000000, 0.000000000000000000, 19.50000000000000000 ) ) ;
#4751=COLOUR_RGB('Off White',0.89,0.88,0.83);
#4752=FILL_AREA_STYLE_COLOUR('',#4751);
#4753=FILL_AREA_STYLE('',(#4752));
#4754=SURFACE_STYLE_FILL_AREA(#4753);
#4755=SURFACE_SIDE_STYLE('',(#4754));
#4756=SURFACE_STYLE_USAGE(.BOTH.,#4755);
#4757=PRESENTATION_STYLE_ASSIGNMENT((#4756));
ENDSEC;
END-ISO-10303-21;
